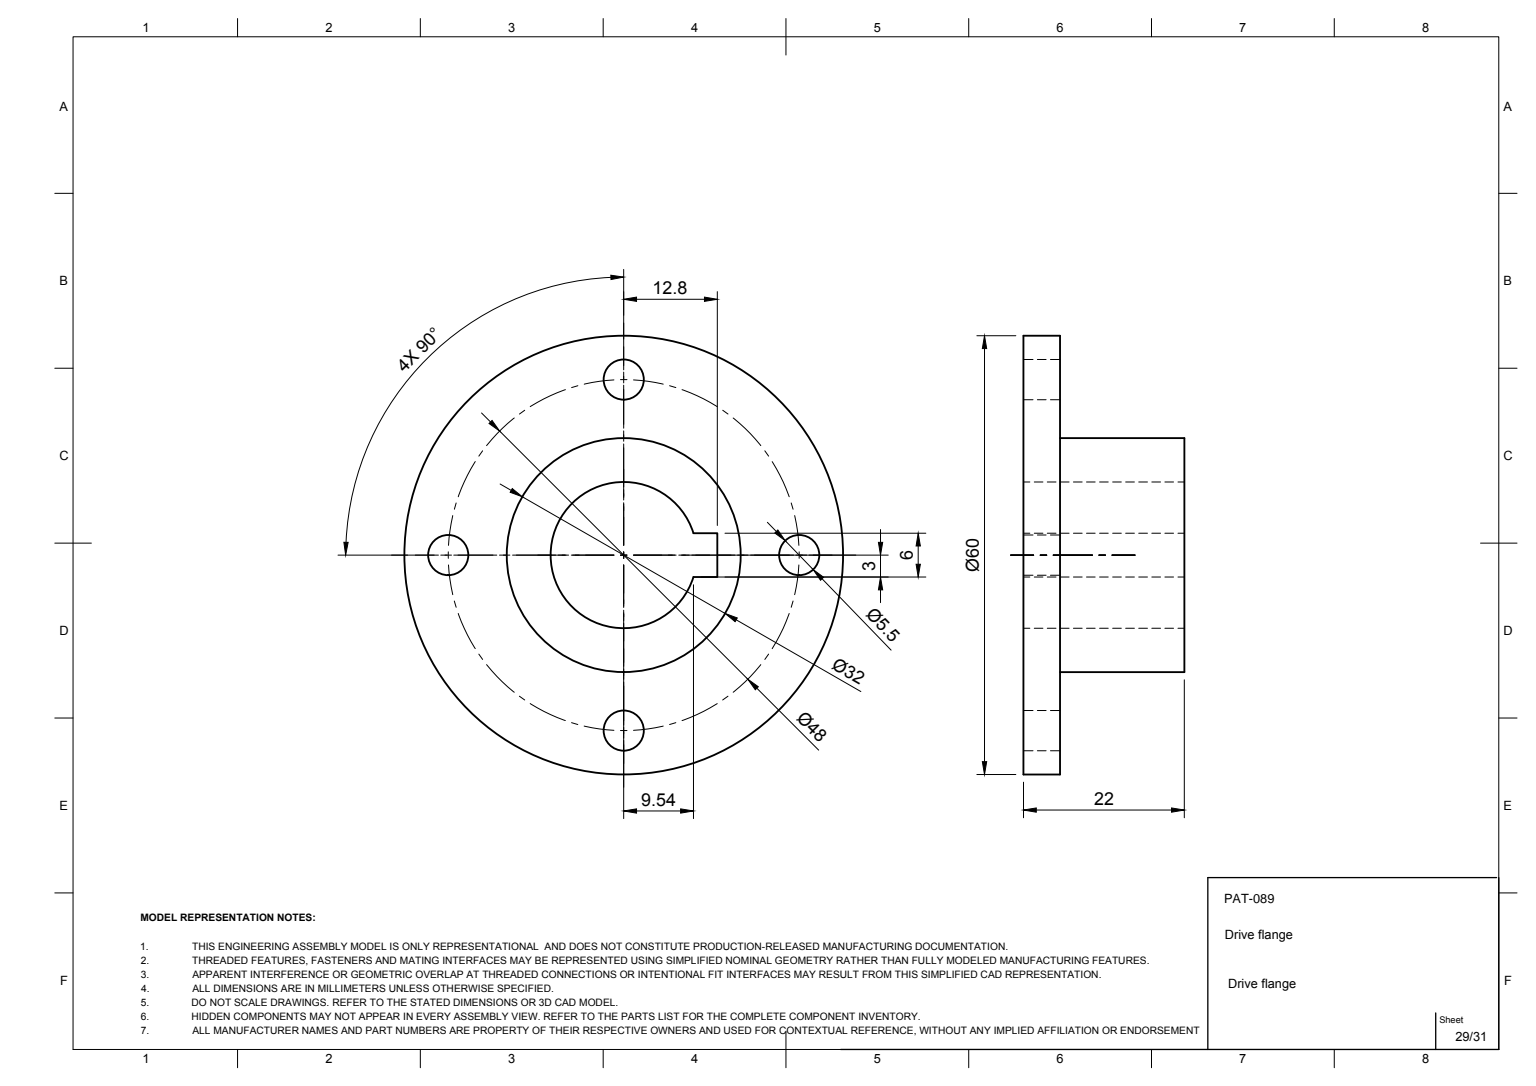
ISO-10303-21;
HEADER;
/* Generated by software containing ST-Developer
 * from STEP Tools, Inc. (www.steptools.com) 
 */

FILE_DESCRIPTION(
/* description */ ('Rotary union on bearing shaft'),
/* implementation_level */ '2;1');

FILE_NAME(
/* name */ 'Drive flange.step',
/* time_stamp */ '2026-10-28T03:24:01-07:00',
/* author */ (''),
/* organization */ (''),
/* preprocessor_version */ 'ST-DEVELOPER v20.2',
/* originating_system */ 'Autodesk Translation Framework v15.17.0.0',
/* authorisation */ '');

FILE_SCHEMA (('AUTOMOTIVE_DESIGN { 1 0 10303 214 3 1 1 }'));
ENDSEC;

DATA;
#10=MECHANICAL_DESIGN_GEOMETRIC_PRESENTATION_REPRESENTATION('',(#342),#9448);
#280=SHAPE_REPRESENTATION_RELATIONSHIP('SRR','None',#9582,#307);
#307=ADVANCED_BREP_SHAPE_REPRESENTATION('',(#375),#9442);
#342=STYLED_ITEM('',(#9771),#375);
#375=MANIFOLD_SOLID_BREP('Body1',#4899);
#468=FACE_BOUND('',#1275,.T.);
#469=FACE_BOUND('',#1276,.T.);
#470=FACE_BOUND('',#1277,.T.);
#471=FACE_BOUND('',#1278,.T.);
#472=FACE_BOUND('',#1279,.T.);
#473=FACE_BOUND('',#1286,.T.);
#474=FACE_BOUND('',#1287,.T.);
#475=FACE_BOUND('',#1288,.T.);
#476=FACE_BOUND('',#1289,.T.);
#477=FACE_BOUND('',#1290,.T.);
#478=FACE_BOUND('',#1294,.T.);
#608=PLANE('',#5677);
#609=PLANE('',#5678);
#610=PLANE('',#5679);
#611=PLANE('',#5680);
#612=PLANE('',#5697);
#613=PLANE('',#5703);
#884=FACE_OUTER_BOUND('',#1271,.T.);
#885=FACE_OUTER_BOUND('',#1272,.T.);
#886=FACE_OUTER_BOUND('',#1273,.T.);
#887=FACE_OUTER_BOUND('',#1274,.T.);
#888=FACE_OUTER_BOUND('',#1280,.T.);
#889=FACE_OUTER_BOUND('',#1281,.T.);
#890=FACE_OUTER_BOUND('',#1282,.T.);
#891=FACE_OUTER_BOUND('',#1283,.T.);
#892=FACE_OUTER_BOUND('',#1284,.T.);
#893=FACE_OUTER_BOUND('',#1285,.T.);
#894=FACE_OUTER_BOUND('',#1291,.T.);
#895=FACE_OUTER_BOUND('',#1292,.T.);
#896=FACE_OUTER_BOUND('',#1293,.T.);
#1271=EDGE_LOOP('',(#4183,#4184,#4185,#4186));
#1272=EDGE_LOOP('',(#4187,#4188,#4189,#4190));
#1273=EDGE_LOOP('',(#4191,#4192,#4193,#4194));
#1274=EDGE_LOOP('',(#4195));
#1275=EDGE_LOOP('',(#4196));
#1276=EDGE_LOOP('',(#4197));
#1277=EDGE_LOOP('',(#4198));
#1278=EDGE_LOOP('',(#4199));
#1279=EDGE_LOOP('',(#4200,#4201,#4202,#4203));
#1280=EDGE_LOOP('',(#4204,#4205,#4206,#4207));
#1281=EDGE_LOOP('',(#4208,#4209,#4210,#4211));
#1282=EDGE_LOOP('',(#4212,#4213,#4214,#4215));
#1283=EDGE_LOOP('',(#4216,#4217,#4218,#4219));
#1284=EDGE_LOOP('',(#4220,#4221,#4222,#4223));
#1285=EDGE_LOOP('',(#4224));
#1286=EDGE_LOOP('',(#4225));
#1287=EDGE_LOOP('',(#4226));
#1288=EDGE_LOOP('',(#4227));
#1289=EDGE_LOOP('',(#4228));
#1290=EDGE_LOOP('',(#4229));
#1291=EDGE_LOOP('',(#4230,#4231,#4232,#4233));
#1292=EDGE_LOOP('',(#4234,#4235,#4236,#4237));
#1293=EDGE_LOOP('',(#4238));
#1294=EDGE_LOOP('',(#4239,#4240,#4241,#4242));
#1571=LINE('',#9031,#1891);
#1572=LINE('',#9033,#1892);
#1573=LINE('',#9035,#1893);
#1574=LINE('',#9036,#1894);
#1575=LINE('',#9039,#1895);
#1576=LINE('',#9041,#1896);
#1577=LINE('',#9042,#1897);
#1578=LINE('',#9045,#1898);
#1579=LINE('',#9047,#1899);
#1580=LINE('',#9048,#1900);
#1581=LINE('',#9066,#1901);
#1582=LINE('',#9070,#1902);
#1583=LINE('',#9074,#1903);
#1584=LINE('',#9078,#1904);
#1585=LINE('',#9085,#1905);
#1586=LINE('',#9088,#1906);
#1891=VECTOR('',#6986,1.);
#1892=VECTOR('',#6987,1.);
#1893=VECTOR('',#6988,1.);
#1894=VECTOR('',#6989,1.);
#1895=VECTOR('',#6992,1.);
#1896=VECTOR('',#6993,1.);
#1897=VECTOR('',#6994,1.);
#1898=VECTOR('',#6997,1.);
#1899=VECTOR('',#6998,1.);
#1900=VECTOR('',#6999,1.);
#1901=VECTOR('',#7022,0.275);
#1902=VECTOR('',#7027,0.275);
#1903=VECTOR('',#7032,0.275);
#1904=VECTOR('',#7037,0.275);
#1905=VECTOR('',#7046,3.);
#1906=VECTOR('',#7049,1.6);
#2215=CIRCLE('',#5681,3.);
#2216=CIRCLE('',#5682,0.275);
#2217=CIRCLE('',#5683,0.275);
#2218=CIRCLE('',#5684,0.275);
#2219=CIRCLE('',#5685,0.275);
#2220=CIRCLE('',#5686,1.);
#2221=CIRCLE('',#5688,1.);
#2222=CIRCLE('',#5690,0.275);
#2223=CIRCLE('',#5692,0.275);
#2224=CIRCLE('',#5694,0.275);
#2225=CIRCLE('',#5696,0.275);
#2226=CIRCLE('',#5698,3.);
#2227=CIRCLE('',#5699,1.6);
#2228=CIRCLE('',#5702,1.6);
#2565=VERTEX_POINT('',#9029);
#2566=VERTEX_POINT('',#9030);
#2567=VERTEX_POINT('',#9032);
#2568=VERTEX_POINT('',#9034);
#2569=VERTEX_POINT('',#9038);
#2570=VERTEX_POINT('',#9040);
#2571=VERTEX_POINT('',#9044);
#2572=VERTEX_POINT('',#9046);
#2573=VERTEX_POINT('',#9050);
#2574=VERTEX_POINT('',#9052);
#2575=VERTEX_POINT('',#9054);
#2576=VERTEX_POINT('',#9056);
#2577=VERTEX_POINT('',#9058);
#2578=VERTEX_POINT('',#9064);
#2579=VERTEX_POINT('',#9068);
#2580=VERTEX_POINT('',#9072);
#2581=VERTEX_POINT('',#9076);
#2582=VERTEX_POINT('',#9080);
#2583=VERTEX_POINT('',#9082);
#2584=VERTEX_POINT('',#9087);
#3119=EDGE_CURVE('',#2565,#2566,#1571,.T.);
#3120=EDGE_CURVE('',#2565,#2567,#1572,.T.);
#3121=EDGE_CURVE('',#2568,#2567,#1573,.T.);
#3122=EDGE_CURVE('',#2566,#2568,#1574,.T.);
#3123=EDGE_CURVE('',#2569,#2565,#1575,.T.);
#3124=EDGE_CURVE('',#2569,#2570,#1576,.T.);
#3125=EDGE_CURVE('',#2567,#2570,#1577,.T.);
#3126=EDGE_CURVE('',#2571,#2569,#1578,.T.);
#3127=EDGE_CURVE('',#2572,#2571,#1579,.T.);
#3128=EDGE_CURVE('',#2570,#2572,#1580,.T.);
#3129=EDGE_CURVE('',#2573,#2573,#2215,.T.);
#3130=EDGE_CURVE('',#2574,#2574,#2216,.T.);
#3131=EDGE_CURVE('',#2575,#2575,#2217,.T.);
#3132=EDGE_CURVE('',#2576,#2576,#2218,.T.);
#3133=EDGE_CURVE('',#2577,#2577,#2219,.T.);
#3134=EDGE_CURVE('',#2572,#2568,#2220,.T.);
#3135=EDGE_CURVE('',#2571,#2566,#2221,.T.);
#3136=EDGE_CURVE('',#2578,#2578,#2222,.T.);
#3137=EDGE_CURVE('',#2578,#2574,#1581,.T.);
#3138=EDGE_CURVE('',#2579,#2579,#2223,.T.);
#3139=EDGE_CURVE('',#2579,#2575,#1582,.T.);
#3140=EDGE_CURVE('',#2580,#2580,#2224,.T.);
#3141=EDGE_CURVE('',#2580,#2576,#1583,.T.);
#3142=EDGE_CURVE('',#2581,#2581,#2225,.T.);
#3143=EDGE_CURVE('',#2581,#2577,#1584,.T.);
#3144=EDGE_CURVE('',#2582,#2582,#2226,.T.);
#3145=EDGE_CURVE('',#2583,#2583,#2227,.T.);
#3146=EDGE_CURVE('',#2573,#2582,#1585,.T.);
#3147=EDGE_CURVE('',#2583,#2584,#1586,.T.);
#3148=EDGE_CURVE('',#2584,#2584,#2228,.T.);
#4183=ORIENTED_EDGE('',*,*,#3119,.F.);
#4184=ORIENTED_EDGE('',*,*,#3120,.T.);
#4185=ORIENTED_EDGE('',*,*,#3121,.F.);
#4186=ORIENTED_EDGE('',*,*,#3122,.F.);
#4187=ORIENTED_EDGE('',*,*,#3123,.F.);
#4188=ORIENTED_EDGE('',*,*,#3124,.T.);
#4189=ORIENTED_EDGE('',*,*,#3125,.F.);
#4190=ORIENTED_EDGE('',*,*,#3120,.F.);
#4191=ORIENTED_EDGE('',*,*,#3126,.F.);
#4192=ORIENTED_EDGE('',*,*,#3127,.F.);
#4193=ORIENTED_EDGE('',*,*,#3128,.F.);
#4194=ORIENTED_EDGE('',*,*,#3124,.F.);
#4195=ORIENTED_EDGE('',*,*,#3129,.T.);
#4196=ORIENTED_EDGE('',*,*,#3130,.T.);
#4197=ORIENTED_EDGE('',*,*,#3131,.T.);
#4198=ORIENTED_EDGE('',*,*,#3132,.T.);
#4199=ORIENTED_EDGE('',*,*,#3133,.T.);
#4200=ORIENTED_EDGE('',*,*,#3121,.T.);
#4201=ORIENTED_EDGE('',*,*,#3125,.T.);
#4202=ORIENTED_EDGE('',*,*,#3128,.T.);
#4203=ORIENTED_EDGE('',*,*,#3134,.T.);
#4204=ORIENTED_EDGE('',*,*,#3122,.T.);
#4205=ORIENTED_EDGE('',*,*,#3134,.F.);
#4206=ORIENTED_EDGE('',*,*,#3127,.T.);
#4207=ORIENTED_EDGE('',*,*,#3135,.T.);
#4208=ORIENTED_EDGE('',*,*,#3136,.F.);
#4209=ORIENTED_EDGE('',*,*,#3137,.T.);
#4210=ORIENTED_EDGE('',*,*,#3130,.F.);
#4211=ORIENTED_EDGE('',*,*,#3137,.F.);
#4212=ORIENTED_EDGE('',*,*,#3138,.F.);
#4213=ORIENTED_EDGE('',*,*,#3139,.T.);
#4214=ORIENTED_EDGE('',*,*,#3131,.F.);
#4215=ORIENTED_EDGE('',*,*,#3139,.F.);
#4216=ORIENTED_EDGE('',*,*,#3140,.F.);
#4217=ORIENTED_EDGE('',*,*,#3141,.T.);
#4218=ORIENTED_EDGE('',*,*,#3132,.F.);
#4219=ORIENTED_EDGE('',*,*,#3141,.F.);
#4220=ORIENTED_EDGE('',*,*,#3142,.F.);
#4221=ORIENTED_EDGE('',*,*,#3143,.T.);
#4222=ORIENTED_EDGE('',*,*,#3133,.F.);
#4223=ORIENTED_EDGE('',*,*,#3143,.F.);
#4224=ORIENTED_EDGE('',*,*,#3144,.F.);
#4225=ORIENTED_EDGE('',*,*,#3145,.F.);
#4226=ORIENTED_EDGE('',*,*,#3142,.T.);
#4227=ORIENTED_EDGE('',*,*,#3140,.T.);
#4228=ORIENTED_EDGE('',*,*,#3138,.T.);
#4229=ORIENTED_EDGE('',*,*,#3136,.T.);
#4230=ORIENTED_EDGE('',*,*,#3129,.F.);
#4231=ORIENTED_EDGE('',*,*,#3146,.T.);
#4232=ORIENTED_EDGE('',*,*,#3144,.T.);
#4233=ORIENTED_EDGE('',*,*,#3146,.F.);
#4234=ORIENTED_EDGE('',*,*,#3145,.T.);
#4235=ORIENTED_EDGE('',*,*,#3147,.T.);
#4236=ORIENTED_EDGE('',*,*,#3148,.T.);
#4237=ORIENTED_EDGE('',*,*,#3147,.F.);
#4238=ORIENTED_EDGE('',*,*,#3148,.F.);
#4239=ORIENTED_EDGE('',*,*,#3119,.T.);
#4240=ORIENTED_EDGE('',*,*,#3135,.F.);
#4241=ORIENTED_EDGE('',*,*,#3126,.T.);
#4242=ORIENTED_EDGE('',*,*,#3123,.T.);
#4554=CYLINDRICAL_SURFACE('',#5687,1.);
#4555=CYLINDRICAL_SURFACE('',#5689,0.275);
#4556=CYLINDRICAL_SURFACE('',#5691,0.275);
#4557=CYLINDRICAL_SURFACE('',#5693,0.275);
#4558=CYLINDRICAL_SURFACE('',#5695,0.275);
#4559=CYLINDRICAL_SURFACE('',#5700,3.);
#4560=CYLINDRICAL_SURFACE('',#5701,1.6);
#4797=ADVANCED_FACE('',(#884),#608,.F.);
#4798=ADVANCED_FACE('',(#885),#609,.F.);
#4799=ADVANCED_FACE('',(#886),#610,.F.);
#4800=ADVANCED_FACE('',(#887,#468,#469,#470,#471,#472),#611,.T.);
#4801=ADVANCED_FACE('',(#888),#4554,.F.);
#4802=ADVANCED_FACE('',(#889),#4555,.F.);
#4803=ADVANCED_FACE('',(#890),#4556,.F.);
#4804=ADVANCED_FACE('',(#891),#4557,.F.);
#4805=ADVANCED_FACE('',(#892),#4558,.F.);
#4806=ADVANCED_FACE('',(#893,#473,#474,#475,#476,#477),#612,.F.);
#4807=ADVANCED_FACE('',(#894),#4559,.T.);
#4808=ADVANCED_FACE('',(#895),#4560,.T.);
#4809=ADVANCED_FACE('',(#896,#478),#613,.F.);
#4899=CLOSED_SHELL('',(#4797,#4798,#4799,#4800,#4801,#4802,#4803,#4804,
#4805,#4806,#4807,#4808,#4809));
#5676=AXIS2_PLACEMENT_3D('',#9027,#6982,#6983);
#5677=AXIS2_PLACEMENT_3D('',#9028,#6984,#6985);
#5678=AXIS2_PLACEMENT_3D('',#9037,#6990,#6991);
#5679=AXIS2_PLACEMENT_3D('',#9043,#6995,#6996);
#5680=AXIS2_PLACEMENT_3D('',#9049,#7000,#7001);
#5681=AXIS2_PLACEMENT_3D('',#9051,#7002,#7003);
#5682=AXIS2_PLACEMENT_3D('',#9053,#7004,#7005);
#5683=AXIS2_PLACEMENT_3D('',#9055,#7006,#7007);
#5684=AXIS2_PLACEMENT_3D('',#9057,#7008,#7009);
#5685=AXIS2_PLACEMENT_3D('',#9059,#7010,#7011);
#5686=AXIS2_PLACEMENT_3D('',#9060,#7012,#7013);
#5687=AXIS2_PLACEMENT_3D('',#9061,#7014,#7015);
#5688=AXIS2_PLACEMENT_3D('',#9062,#7016,#7017);
#5689=AXIS2_PLACEMENT_3D('',#9063,#7018,#7019);
#5690=AXIS2_PLACEMENT_3D('',#9065,#7020,#7021);
#5691=AXIS2_PLACEMENT_3D('',#9067,#7023,#7024);
#5692=AXIS2_PLACEMENT_3D('',#9069,#7025,#7026);
#5693=AXIS2_PLACEMENT_3D('',#9071,#7028,#7029);
#5694=AXIS2_PLACEMENT_3D('',#9073,#7030,#7031);
#5695=AXIS2_PLACEMENT_3D('',#9075,#7033,#7034);
#5696=AXIS2_PLACEMENT_3D('',#9077,#7035,#7036);
#5697=AXIS2_PLACEMENT_3D('',#9079,#7038,#7039);
#5698=AXIS2_PLACEMENT_3D('',#9081,#7040,#7041);
#5699=AXIS2_PLACEMENT_3D('',#9083,#7042,#7043);
#5700=AXIS2_PLACEMENT_3D('',#9084,#7044,#7045);
#5701=AXIS2_PLACEMENT_3D('',#9086,#7047,#7048);
#5702=AXIS2_PLACEMENT_3D('',#9089,#7050,#7051);
#5703=AXIS2_PLACEMENT_3D('',#9090,#7052,#7053);
#6982=DIRECTION('axis',(0.,0.,1.));
#6983=DIRECTION('refdir',(1.,0.,0.));
#6984=DIRECTION('center_axis',(-1.,0.,0.));
#6985=DIRECTION('ref_axis',(0.,0.,1.));
#6986=DIRECTION('',(0.,0.,1.));
#6987=DIRECTION('',(0.,1.,0.));
#6988=DIRECTION('',(0.,0.,-1.));
#6989=DIRECTION('',(0.,1.,0.));
#6990=DIRECTION('center_axis',(0.,0.,-1.));
#6991=DIRECTION('ref_axis',(-1.,0.,0.));
#6992=DIRECTION('',(-1.,0.,0.));
#6993=DIRECTION('',(0.,1.,0.));
#6994=DIRECTION('',(1.,0.,0.));
#6995=DIRECTION('center_axis',(1.,0.,0.));
#6996=DIRECTION('ref_axis',(0.,0.,-1.));
#6997=DIRECTION('',(0.,0.,-1.));
#6998=DIRECTION('',(0.,-1.,0.));
#6999=DIRECTION('',(0.,0.,1.));
#7000=DIRECTION('center_axis',(0.,1.,0.));
#7001=DIRECTION('ref_axis',(1.,0.,0.));
#7002=DIRECTION('center_axis',(0.,1.,0.));
#7003=DIRECTION('ref_axis',(1.,0.,0.));
#7004=DIRECTION('center_axis',(0.,-1.,0.));
#7005=DIRECTION('ref_axis',(1.,0.,0.));
#7006=DIRECTION('center_axis',(0.,-1.,0.));
#7007=DIRECTION('ref_axis',(1.,0.,0.));
#7008=DIRECTION('center_axis',(0.,-1.,0.));
#7009=DIRECTION('ref_axis',(1.,0.,0.));
#7010=DIRECTION('center_axis',(0.,-1.,0.));
#7011=DIRECTION('ref_axis',(1.,0.,0.));
#7012=DIRECTION('center_axis',(0.,-1.,0.));
#7013=DIRECTION('ref_axis',(1.,0.,0.));
#7014=DIRECTION('center_axis',(0.,1.,0.));
#7015=DIRECTION('ref_axis',(-1.83697019872103E-16,0.,1.));
#7016=DIRECTION('center_axis',(0.,-1.,0.));
#7017=DIRECTION('ref_axis',(1.,0.,0.));
#7018=DIRECTION('center_axis',(0.,1.,0.));
#7019=DIRECTION('ref_axis',(1.,0.,0.));
#7020=DIRECTION('center_axis',(0.,1.,0.));
#7021=DIRECTION('ref_axis',(1.,0.,0.));
#7022=DIRECTION('',(0.,1.,0.));
#7023=DIRECTION('center_axis',(0.,1.,0.));
#7024=DIRECTION('ref_axis',(1.,0.,0.));
#7025=DIRECTION('center_axis',(0.,1.,0.));
#7026=DIRECTION('ref_axis',(1.,0.,0.));
#7027=DIRECTION('',(0.,1.,0.));
#7028=DIRECTION('center_axis',(0.,1.,0.));
#7029=DIRECTION('ref_axis',(1.,0.,0.));
#7030=DIRECTION('center_axis',(0.,1.,0.));
#7031=DIRECTION('ref_axis',(1.,0.,0.));
#7032=DIRECTION('',(0.,1.,0.));
#7033=DIRECTION('center_axis',(0.,1.,0.));
#7034=DIRECTION('ref_axis',(1.,0.,0.));
#7035=DIRECTION('center_axis',(0.,1.,0.));
#7036=DIRECTION('ref_axis',(1.,0.,0.));
#7037=DIRECTION('',(0.,1.,0.));
#7038=DIRECTION('center_axis',(0.,1.,0.));
#7039=DIRECTION('ref_axis',(1.,0.,0.));
#7040=DIRECTION('center_axis',(0.,1.,0.));
#7041=DIRECTION('ref_axis',(1.,0.,0.));
#7042=DIRECTION('center_axis',(0.,-1.,0.));
#7043=DIRECTION('ref_axis',(1.,0.,0.));
#7044=DIRECTION('center_axis',(0.,1.,0.));
#7045=DIRECTION('ref_axis',(1.,0.,0.));
#7046=DIRECTION('',(0.,-1.,0.));
#7047=DIRECTION('center_axis',(0.,1.,0.));
#7048=DIRECTION('ref_axis',(1.,0.,0.));
#7049=DIRECTION('',(0.,-1.,0.));
#7050=DIRECTION('center_axis',(0.,1.,0.));
#7051=DIRECTION('ref_axis',(1.,0.,0.));
#7052=DIRECTION('center_axis',(0.,1.,0.));
#7053=DIRECTION('ref_axis',(1.,0.,0.));
#9027=CARTESIAN_POINT('',(0.,0.,0.));
#9028=CARTESIAN_POINT('Origin',(-0.3,7.7,3.22));
#9029=CARTESIAN_POINT('',(-0.3,7.8,3.22));
#9030=CARTESIAN_POINT('',(-0.3,7.8,3.54606079858305));
#9031=CARTESIAN_POINT('',(-0.3,7.8,3.86));
#9032=CARTESIAN_POINT('',(-0.3,10.,3.22));
#9033=CARTESIAN_POINT('',(-0.3,7.7,3.22));
#9034=CARTESIAN_POINT('',(-0.3,10.,3.54606079858305));
#9035=CARTESIAN_POINT('',(-0.3,10.,3.86));
#9036=CARTESIAN_POINT('',(-0.3,7.8,3.54606079858305));
#9037=CARTESIAN_POINT('Origin',(0.3,7.7,3.22));
#9038=CARTESIAN_POINT('',(0.3,7.8,3.22));
#9039=CARTESIAN_POINT('',(0.15,7.8,3.22));
#9040=CARTESIAN_POINT('',(0.3,10.,3.22));
#9041=CARTESIAN_POINT('',(0.3,7.7,3.22));
#9042=CARTESIAN_POINT('',(0.15,10.,3.22));
#9043=CARTESIAN_POINT('Origin',(0.3,7.7,4.5));
#9044=CARTESIAN_POINT('',(0.3,7.8,3.54606079858305));
#9045=CARTESIAN_POINT('',(0.3,7.8,4.5));
#9046=CARTESIAN_POINT('',(0.3,10.,3.54606079858305));
#9047=CARTESIAN_POINT('',(0.3,7.8,3.54606079858305));
#9048=CARTESIAN_POINT('',(0.3,10.,4.5));
#9049=CARTESIAN_POINT('Origin',(0.,10.,4.5));
#9050=CARTESIAN_POINT('',(-3.,10.,4.5));
#9051=CARTESIAN_POINT('Origin',(0.,10.,4.5));
#9052=CARTESIAN_POINT('',(-2.675,10.,4.5));
#9053=CARTESIAN_POINT('Origin',(-2.4,10.,4.5));
#9054=CARTESIAN_POINT('',(-0.275,10.,6.9));
#9055=CARTESIAN_POINT('Origin',(1.46957615897682E-16,10.,6.9));
#9056=CARTESIAN_POINT('',(2.125,10.,4.5));
#9057=CARTESIAN_POINT('Origin',(2.4,10.,4.5));
#9058=CARTESIAN_POINT('',(-0.275,10.,2.1));
#9059=CARTESIAN_POINT('Origin',(-4.40872847693047E-16,10.,2.1));
#9060=CARTESIAN_POINT('Origin',(0.,10.,4.5));
#9061=CARTESIAN_POINT('Origin',(0.,7.8,4.5));
#9062=CARTESIAN_POINT('Origin',(0.,7.8,4.5));
#9063=CARTESIAN_POINT('Origin',(-2.4,9.4,4.5));
#9064=CARTESIAN_POINT('',(-2.675,9.5,4.5));
#9065=CARTESIAN_POINT('Origin',(-2.4,9.5,4.5));
#9066=CARTESIAN_POINT('',(-2.675,9.4,4.5));
#9067=CARTESIAN_POINT('Origin',(1.46957615897682E-16,9.4,6.9));
#9068=CARTESIAN_POINT('',(-0.275,9.5,6.9));
#9069=CARTESIAN_POINT('Origin',(1.46957615897682E-16,9.5,6.9));
#9070=CARTESIAN_POINT('',(-0.275,9.4,6.9));
#9071=CARTESIAN_POINT('Origin',(2.4,9.4,4.5));
#9072=CARTESIAN_POINT('',(2.125,9.5,4.5));
#9073=CARTESIAN_POINT('Origin',(2.4,9.5,4.5));
#9074=CARTESIAN_POINT('',(2.125,9.4,4.5));
#9075=CARTESIAN_POINT('Origin',(-4.40872847693047E-16,9.4,2.1));
#9076=CARTESIAN_POINT('',(-0.275,9.5,2.1));
#9077=CARTESIAN_POINT('Origin',(-4.40872847693047E-16,9.5,2.1));
#9078=CARTESIAN_POINT('',(-0.275,9.4,2.1));
#9079=CARTESIAN_POINT('Origin',(0.,9.5,4.5));
#9080=CARTESIAN_POINT('',(-3.,9.5,4.5));
#9081=CARTESIAN_POINT('Origin',(0.,9.5,4.5));
#9082=CARTESIAN_POINT('',(-1.6,9.5,4.5));
#9083=CARTESIAN_POINT('Origin',(0.,9.5,4.5));
#9084=CARTESIAN_POINT('Origin',(0.,9.5,4.5));
#9085=CARTESIAN_POINT('',(-3.,9.5,4.5));
#9086=CARTESIAN_POINT('Origin',(0.,7.8,4.5));
#9087=CARTESIAN_POINT('',(-1.6,7.8,4.5));
#9088=CARTESIAN_POINT('',(-1.6,7.8,4.5));
#9089=CARTESIAN_POINT('Origin',(0.,7.8,4.5));
#9090=CARTESIAN_POINT('Origin',(0.,7.8,4.5));
#9410=UNCERTAINTY_MEASURE_WITH_UNIT(LENGTH_MEASURE(0.001),#9449,
'DISTANCE_ACCURACY_VALUE',
'Maximum model space distance between geometric entities at asserted c
onnectivities');
#9416=UNCERTAINTY_MEASURE_WITH_UNIT(LENGTH_MEASURE(0.001),#9449,
'DISTANCE_ACCURACY_VALUE',
'Maximum model space distance between geometric entities at asserted c
onnectivities');
#9442=(
GEOMETRIC_REPRESENTATION_CONTEXT(3)
GLOBAL_UNCERTAINTY_ASSIGNED_CONTEXT((#9410))
GLOBAL_UNIT_ASSIGNED_CONTEXT((#9449,#9451,#9452))
REPRESENTATION_CONTEXT('','3D')
);
#9448=(
GEOMETRIC_REPRESENTATION_CONTEXT(3)
GLOBAL_UNCERTAINTY_ASSIGNED_CONTEXT((#9416))
GLOBAL_UNIT_ASSIGNED_CONTEXT((#9449,#9451,#9452))
REPRESENTATION_CONTEXT('','3D')
);
#9449=(
LENGTH_UNIT()
NAMED_UNIT(*)
SI_UNIT(.CENTI.,.METRE.)
);
#9451=(
NAMED_UNIT(*)
PLANE_ANGLE_UNIT()
SI_UNIT($,.RADIAN.)
);
#9452=(
NAMED_UNIT(*)
SI_UNIT($,.STERADIAN.)
SOLID_ANGLE_UNIT()
);
#9478=SHAPE_DEFINITION_REPRESENTATION(#9514,#9582);
#9514=PRODUCT_DEFINITION_SHAPE('',$,#9614);
#9582=SHAPE_REPRESENTATION('',(#5676),#9442);
#9588=PRODUCT_DEFINITION_CONTEXT('part definition',#9683,'design');
#9614=PRODUCT_DEFINITION('Drive flange','Drive flange',#9645,#9588);
#9645=PRODUCT_DEFINITION_FORMATION('',$,#9710);
#9683=APPLICATION_CONTEXT(
'Core Data for Automotive Mechanical Design Process');
#9684=PRODUCT_CONTEXT('part definition',#9683,'mechanical');
#9710=PRODUCT('Drive flange','Drive flange','Drive flange',(#9684));
#9765=COLOUR_RGB('Sky Blue',0.24,0.69,0.87);
#9766=FILL_AREA_STYLE_COLOUR('',#9765);
#9767=FILL_AREA_STYLE('',(#9766));
#9768=SURFACE_STYLE_FILL_AREA(#9767);
#9769=SURFACE_SIDE_STYLE('',(#9768));
#9770=SURFACE_STYLE_USAGE(.BOTH.,#9769);
#9771=PRESENTATION_STYLE_ASSIGNMENT((#9770));
ENDSEC;
END-ISO-10303-21;
